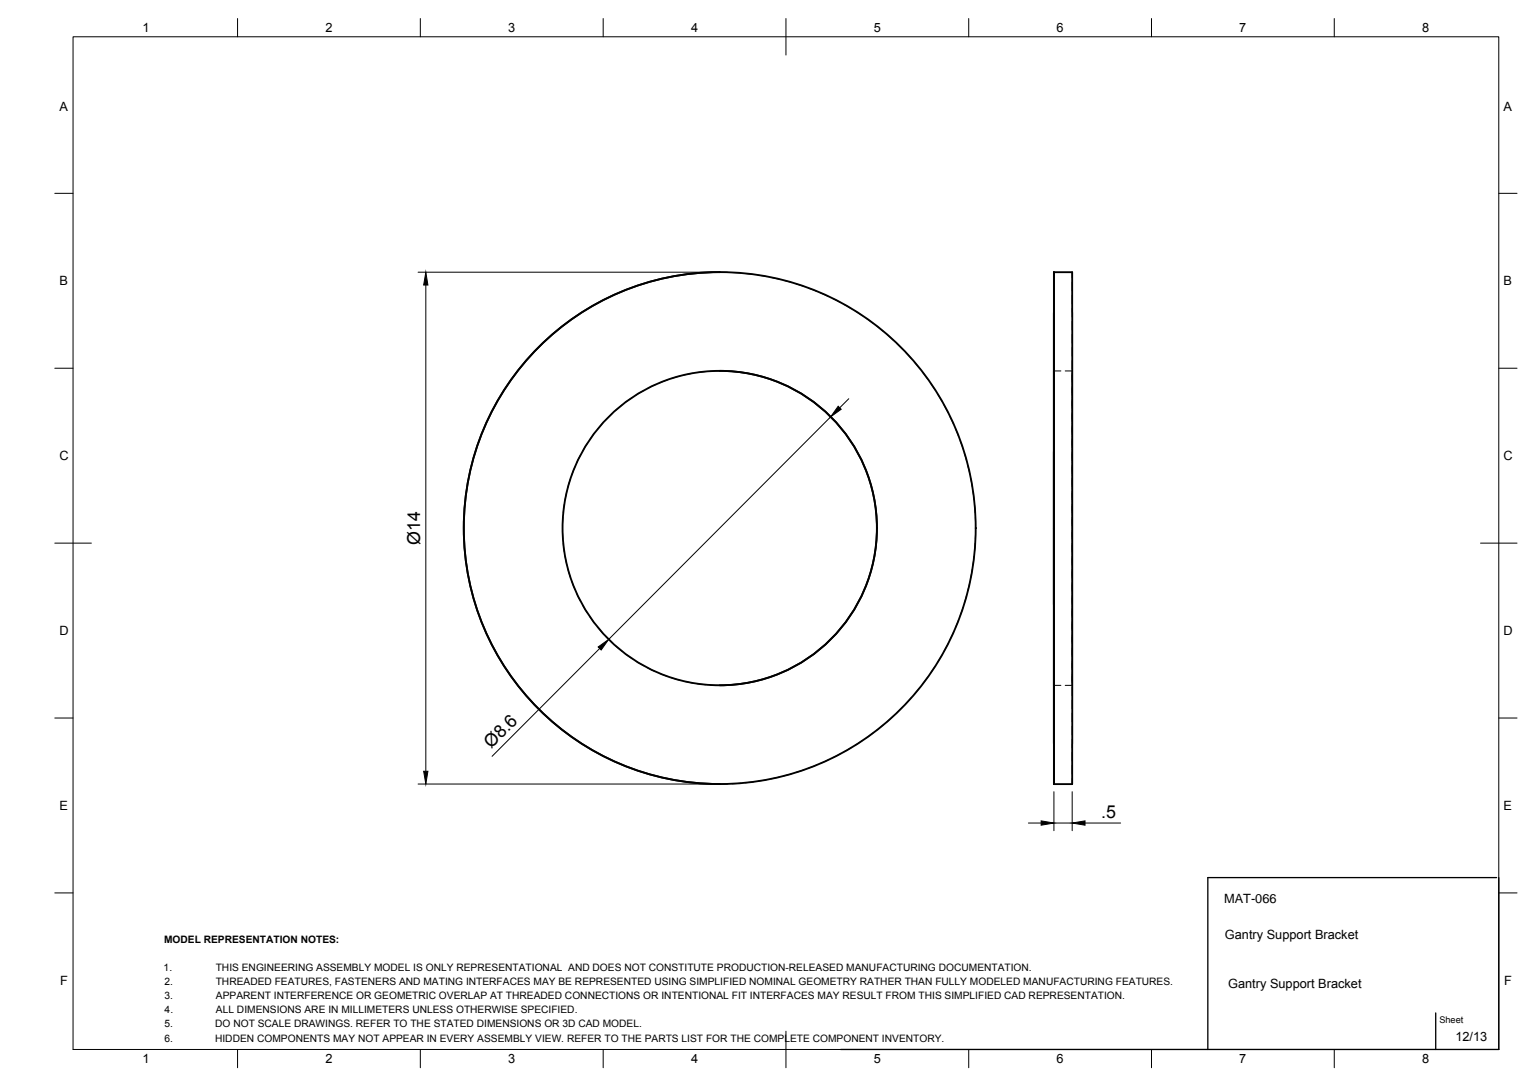
ISO-10303-21;
HEADER;
/* Generated by software containing ST-Developer
 * from STEP Tools, Inc. (www.steptools.com) 
 */

FILE_DESCRIPTION(
/* description */ ('CAx-IF Rec.Pracs.---Representation and Presentation of Product Manufa
cturing Information (PMI)---4.0---2014-10-13'),
/* implementation_level */ '2;1');

FILE_NAME(
/* name */ 'Gantry Support Bracket.step',
/* time_stamp */ '2026-10-24T15:58:00-07:00',
/* author */ (''),
/* organization */ (''),
/* preprocessor_version */ 'ST-DEVELOPER v20.2',
/* originating_system */ 'Autodesk Translation Framework v15.17.0.0',
/* authorisation */ '');

FILE_SCHEMA (('AP242_MANAGED_MODEL_BASED_3D_ENGINEERING_MIM_LF { 1 0 10303 442 2 1 4 }'));
ENDSEC;

DATA;
#10=MECHANICAL_DESIGN_GEOMETRIC_PRESENTATION_REPRESENTATION('',(#136),#8944);
#118=SHAPE_REPRESENTATION_RELATIONSHIP('SRR','None',#9001,#127);
#127=ADVANCED_BREP_SHAPE_REPRESENTATION('',(#145),#8942);
#136=STYLED_ITEM('',(#9054),#145);
#145=MANIFOLD_SOLID_BREP('Body1',#5157);
#234=CYLINDRICAL_SURFACE('',#5775,0.007);
#235=CYLINDRICAL_SURFACE('',#5779,0.0043);
#303=FACE_BOUND('',#901,.T.);
#304=FACE_BOUND('',#904,.T.);
#566=FACE_OUTER_BOUND('',#900,.T.);
#567=FACE_OUTER_BOUND('',#902,.T.);
#568=FACE_OUTER_BOUND('',#903,.T.);
#569=FACE_OUTER_BOUND('',#905,.T.);
#900=EDGE_LOOP('',(#4675));
#901=EDGE_LOOP('',(#4676));
#902=EDGE_LOOP('',(#4677,#4678,#4679,#4680));
#903=EDGE_LOOP('',(#4681));
#904=EDGE_LOOP('',(#4682));
#905=EDGE_LOOP('',(#4683,#4684,#4685,#4686));
#1161=CIRCLE('',#5773,0.00700000000001);
#1162=CIRCLE('',#5774,0.00430000000001);
#1163=CIRCLE('',#5776,0.00700000000001);
#1164=CIRCLE('',#5778,0.00430000000001);
#1621=LINE('',#8866,#2076);
#1622=LINE('',#8872,#2077);
#2076=VECTOR('',#7300,0.007);
#2077=VECTOR('',#7309,0.0043);
#2547=VERTEX_POINT('',#8860);
#2548=VERTEX_POINT('',#8862);
#2549=VERTEX_POINT('',#8865);
#2550=VERTEX_POINT('',#8869);
#3258=EDGE_CURVE('',#2547,#2547,#1161,.T.);
#3259=EDGE_CURVE('',#2548,#2548,#1162,.T.);
#3260=EDGE_CURVE('',#2547,#2549,#1621,.T.);
#3261=EDGE_CURVE('',#2549,#2549,#1163,.T.);
#3262=EDGE_CURVE('',#2550,#2550,#1164,.T.);
#3263=EDGE_CURVE('',#2550,#2548,#1622,.T.);
#4675=ORIENTED_EDGE('',*,*,#3258,.T.);
#4676=ORIENTED_EDGE('',*,*,#3259,.F.);
#4677=ORIENTED_EDGE('',*,*,#3258,.F.);
#4678=ORIENTED_EDGE('',*,*,#3260,.T.);
#4679=ORIENTED_EDGE('',*,*,#3261,.T.);
#4680=ORIENTED_EDGE('',*,*,#3260,.F.);
#4681=ORIENTED_EDGE('',*,*,#3261,.F.);
#4682=ORIENTED_EDGE('',*,*,#3262,.T.);
#4683=ORIENTED_EDGE('',*,*,#3262,.F.);
#4684=ORIENTED_EDGE('',*,*,#3263,.T.);
#4685=ORIENTED_EDGE('',*,*,#3259,.T.);
#4686=ORIENTED_EDGE('',*,*,#3263,.F.);
#4876=PLANE('',#5772);
#4877=PLANE('',#5777);
#5139=ADVANCED_FACE('',(#566,#303),#4876,.F.);
#5140=ADVANCED_FACE('',(#567),#234,.T.);
#5141=ADVANCED_FACE('',(#568,#304),#4877,.F.);
#5142=ADVANCED_FACE('',(#569),#235,.F.);
#5157=CLOSED_SHELL('',(#5139,#5140,#5141,#5142));
#5771=AXIS2_PLACEMENT_3D('',#8858,#7290,#7291);
#5772=AXIS2_PLACEMENT_3D('',#8859,#7292,#7293);
#5773=AXIS2_PLACEMENT_3D('',#8861,#7294,#7295);
#5774=AXIS2_PLACEMENT_3D('',#8863,#7296,#7297);
#5775=AXIS2_PLACEMENT_3D('',#8864,#7298,#7299);
#5776=AXIS2_PLACEMENT_3D('',#8867,#7301,#7302);
#5777=AXIS2_PLACEMENT_3D('',#8868,#7303,#7304);
#5778=AXIS2_PLACEMENT_3D('',#8870,#7305,#7306);
#5779=AXIS2_PLACEMENT_3D('',#8871,#7307,#7308);
#7290=DIRECTION('axis',(0.,0.,1.));
#7291=DIRECTION('refdir',(1.,0.,0.));
#7292=DIRECTION('center_axis',(0.,-1.,0.));
#7293=DIRECTION('ref_axis',(1.,0.,0.));
#7294=DIRECTION('center_axis',(0.,1.,0.));
#7295=DIRECTION('ref_axis',(1.,0.,0.));
#7296=DIRECTION('center_axis',(0.,1.,0.));
#7297=DIRECTION('ref_axis',(1.,0.,0.));
#7298=DIRECTION('center_axis',(0.,1.,0.));
#7299=DIRECTION('ref_axis',(0.,0.,1.));
#7300=DIRECTION('',(0.,-1.,0.));
#7301=DIRECTION('center_axis',(0.,1.,0.));
#7302=DIRECTION('ref_axis',(1.,0.,0.));
#7303=DIRECTION('center_axis',(0.,1.,0.));
#7304=DIRECTION('ref_axis',(0.,0.,1.));
#7305=DIRECTION('center_axis',(0.,1.,0.));
#7306=DIRECTION('ref_axis',(1.,0.,0.));
#7307=DIRECTION('center_axis',(0.,1.,0.));
#7308=DIRECTION('ref_axis',(0.,0.,1.));
#7309=DIRECTION('',(0.,1.,0.));
#8858=CARTESIAN_POINT('',(0.,0.,0.));
#8859=CARTESIAN_POINT('Origin',(0.,0.0109999997541308,0.00699999995096662));
#8860=CARTESIAN_POINT('',(-8.57252759403147E-19,0.0109999997541408,-0.00700000004903339));
#8861=CARTESIAN_POINT('Origin',(0.,0.0109999997541408,-4.90433850849834E-11));
#8862=CARTESIAN_POINT('',(-5.26598123633362E-19,0.0109999997541408,-0.00430000004903338));
#8863=CARTESIAN_POINT('Origin',(0.,0.0109999997541408,-4.90433850849834E-11));
#8864=CARTESIAN_POINT('Origin',(0.,0.0107499997597188,-4.90333850849834E-11));
#8865=CARTESIAN_POINT('',(-8.57252759403147E-19,0.0104999997653167,-0.00700000004903339));
#8866=CARTESIAN_POINT('',(-8.57252759403147E-19,0.0107499997597188,-0.00700000004903339));
#8867=CARTESIAN_POINT('Origin',(0.,0.0104999997653167,-4.90433850849834E-11));
#8868=CARTESIAN_POINT('Origin',(0.,0.0104999997653067,0.00429999995096661));
#8869=CARTESIAN_POINT('',(-5.26598123633362E-19,0.0104999997653167,-0.00430000004903338));
#8870=CARTESIAN_POINT('Origin',(0.,0.0104999997653167,-4.90433850849834E-11));
#8871=CARTESIAN_POINT('Origin',(0.,0.0107499997597188,-4.90333850849834E-11));
#8872=CARTESIAN_POINT('',(-5.26598123633362E-19,0.0107499997597188,-0.00430000004903338));
#8930=UNCERTAINTY_MEASURE_WITH_UNIT(LENGTH_MEASURE(1.E-5),#8945,
'DISTANCE_ACCURACY_VALUE',
'Maximum model space distance between geometric entities at asserted c
onnectivities');
#8932=UNCERTAINTY_MEASURE_WITH_UNIT(LENGTH_MEASURE(1.E-5),#8945,
'DISTANCE_ACCURACY_VALUE',
'Maximum model space distance between geometric entities at asserted c
onnectivities');
#8942=(
GEOMETRIC_REPRESENTATION_CONTEXT(3)
GLOBAL_UNCERTAINTY_ASSIGNED_CONTEXT((#8930))
GLOBAL_UNIT_ASSIGNED_CONTEXT((#8945,#8946,#8947))
REPRESENTATION_CONTEXT('','3D')
);
#8944=(
GEOMETRIC_REPRESENTATION_CONTEXT(3)
GLOBAL_UNCERTAINTY_ASSIGNED_CONTEXT((#8932))
GLOBAL_UNIT_ASSIGNED_CONTEXT((#8945,#8946,#8947))
REPRESENTATION_CONTEXT('','3D')
);
#8945=(
LENGTH_UNIT()
NAMED_UNIT(*)
SI_UNIT($,.METRE.)
);
#8946=(
NAMED_UNIT(*)
PLANE_ANGLE_UNIT()
SI_UNIT($,.RADIAN.)
);
#8947=(
NAMED_UNIT(*)
SI_UNIT($,.STERADIAN.)
SOLID_ANGLE_UNIT()
);
#8957=SHAPE_DEFINITION_REPRESENTATION(#8968,#9001);
#8968=PRODUCT_DEFINITION_SHAPE('',$,#9013);
#9001=SHAPE_REPRESENTATION('',(#5771),#8942);
#9003=PRODUCT_DEFINITION_CONTEXT('part definition',#9038,'design');
#9013=PRODUCT_DEFINITION('Gantry Support Bracket',
'Gantry Support Bracket',#9024,#9003);
#9024=PRODUCT_DEFINITION_FORMATION('',$,#9049);
#9038=APPLICATION_CONTEXT('Managed model based 3d engineering');
#9039=PRODUCT_CONTEXT('part definition',#9038,'mechanical');
#9049=PRODUCT('Gantry Support Bracket','Gantry Support Bracket',
'LEGAL AND USAGE DISCLAIMER: this Data/Model is provided \X2\201C\X0\A
S IS\X2\201D\X0\ for informational and representational only. It is a 
geometric approximation and is NOT engineered, certified, or guarantee
d for dimensional accuracy, exact tolerances, or production-level prec
ision. Vendor disclaims all implied warranties including fitness for a
 particular purpose. DO NOT USE FOR DIRECT PHYSICAL MANUFACTURING, AUT
OMATED PRODUCTION, OR SAFETY-CRITICAL SYSTEMS without independent engi
neering verification and resolution of any design discrepancies.',(#9039));
#9054=PRESENTATION_STYLE_ASSIGNMENT((#9059));
#9059=SURFACE_STYLE_USAGE(.BOTH.,#9064);
#9064=SURFACE_SIDE_STYLE('',(#9069));
#9069=SURFACE_STYLE_FILL_AREA(#9074);
#9074=FILL_AREA_STYLE('Opaque(137,137,137)',(#9079));
#9079=FILL_AREA_STYLE_COLOUR('Opaque(137,137,137)',#9084);
#9084=COLOUR_RGB('Opaque(137,137,137)',0.537254901960784,0.537254901960784,
0.537254901960784);
ENDSEC;
END-ISO-10303-21;
